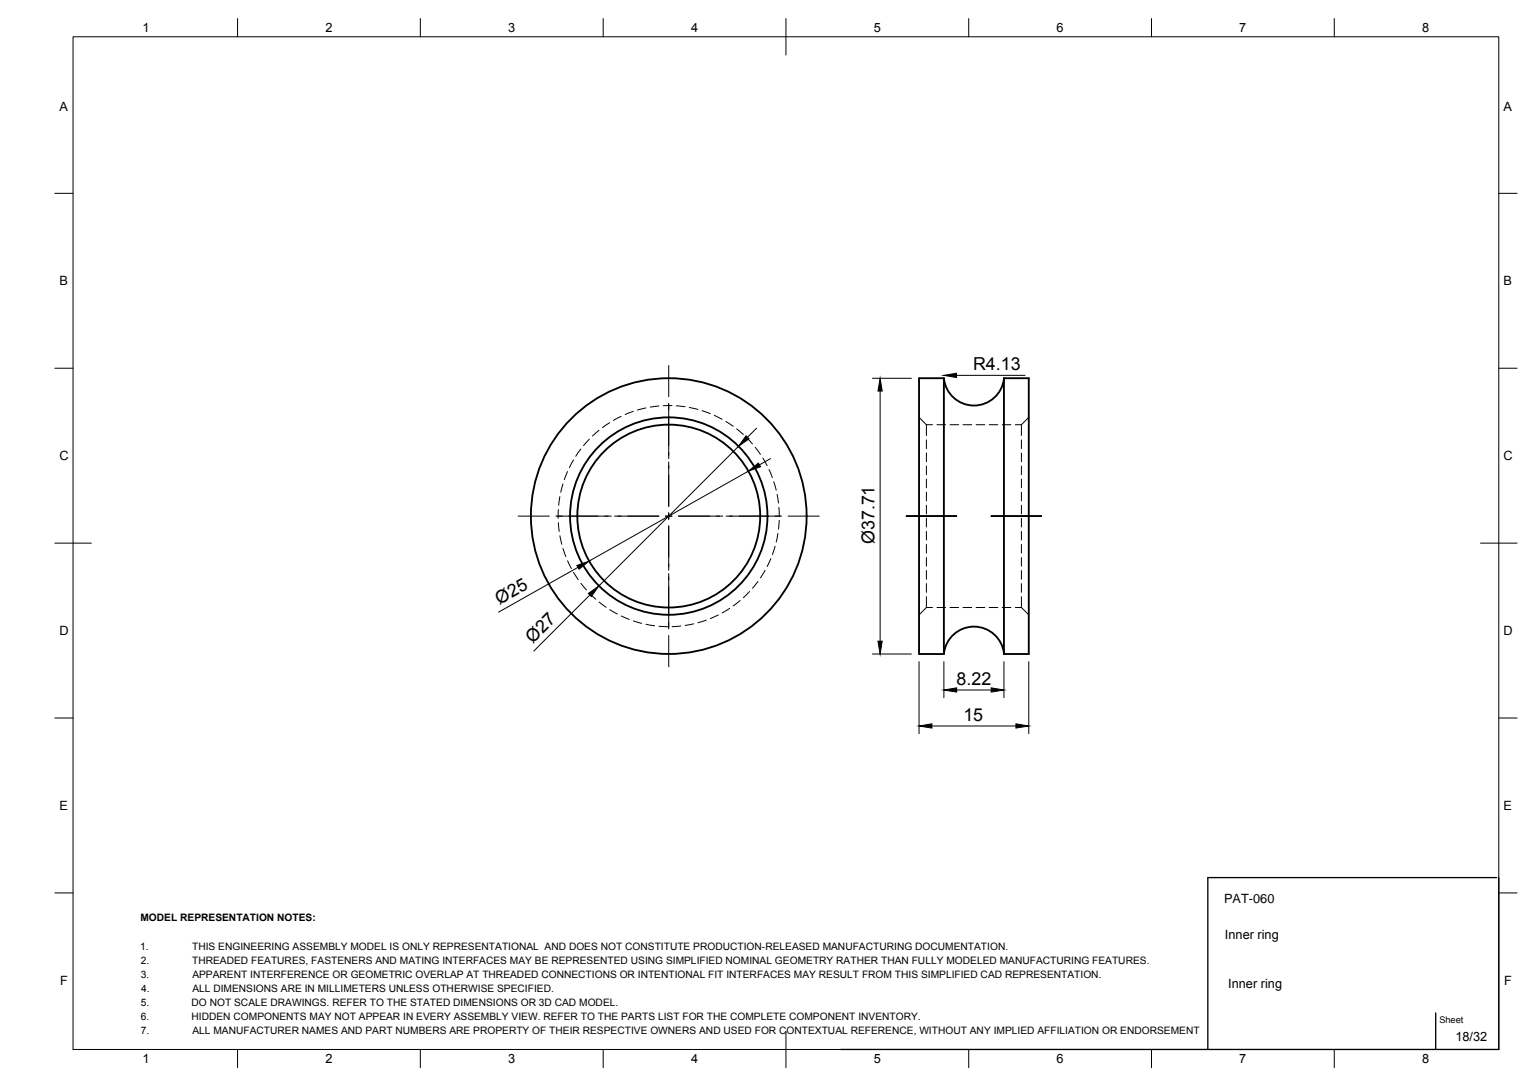
ISO-10303-21;
HEADER;
/* Generated by software containing ST-Developer
 * from STEP Tools, Inc. (www.steptools.com) 
 */

FILE_DESCRIPTION(
/* description */ ('Indexing fixture plate with plunger'),
/* implementation_level */ '2;1');

FILE_NAME(
/* name */ 'Inner ring.step',
/* time_stamp */ '2026-10-28T03:23:41-07:00',
/* author */ (''),
/* organization */ (''),
/* preprocessor_version */ 'ST-DEVELOPER v20.2',
/* originating_system */ 'Autodesk Translation Framework v15.17.0.0',
/* authorisation */ '');

FILE_SCHEMA (('AUTOMOTIVE_DESIGN { 1 0 10303 214 3 1 1 }'));
ENDSEC;

DATA;
#10=MECHANICAL_DESIGN_GEOMETRIC_PRESENTATION_REPRESENTATION('',(#330),#10020);
#213=TOROIDAL_SURFACE('',#5086,1.925,0.412776);
#218=CONICAL_SURFACE('',#5097,1.3,0.785398163397449);
#219=CONICAL_SURFACE('',#5104,1.3,0.785398163397449);
#276=SHAPE_REPRESENTATION_RELATIONSHIP('SRR','None',#10151,#303);
#303=ADVANCED_BREP_SHAPE_REPRESENTATION('',(#365),#10004);
#330=STYLED_ITEM('',(#10368),#365);
#365=MANIFOLD_SOLID_BREP('Body1',#4585);
#431=FACE_BOUND('',#1091,.T.);
#432=FACE_BOUND('',#1094,.T.);
#583=PLANE('',#5099);
#584=PLANE('',#5102);
#756=FACE_OUTER_BOUND('',#1086,.T.);
#757=FACE_OUTER_BOUND('',#1087,.T.);
#758=FACE_OUTER_BOUND('',#1088,.T.);
#759=FACE_OUTER_BOUND('',#1089,.T.);
#760=FACE_OUTER_BOUND('',#1090,.T.);
#761=FACE_OUTER_BOUND('',#1092,.T.);
#762=FACE_OUTER_BOUND('',#1093,.T.);
#763=FACE_OUTER_BOUND('',#1095,.T.);
#1086=EDGE_LOOP('',(#3371,#3372,#3373,#3374,#3375,#3376));
#1087=EDGE_LOOP('',(#3377,#3378,#3379,#3380,#3381));
#1088=EDGE_LOOP('',(#3382,#3383,#3384,#3385));
#1089=EDGE_LOOP('',(#3386,#3387,#3388,#3389));
#1090=EDGE_LOOP('',(#3390));
#1091=EDGE_LOOP('',(#3391));
#1092=EDGE_LOOP('',(#3392,#3393,#3394,#3395,#3396));
#1093=EDGE_LOOP('',(#3397));
#1094=EDGE_LOOP('',(#3398));
#1095=EDGE_LOOP('',(#3399,#3400,#3401,#3402));
#1463=LINE('',#8611,#1683);
#1464=LINE('',#8617,#1684);
#1465=LINE('',#8621,#1685);
#1466=LINE('',#8627,#1686);
#1467=LINE('',#8632,#1687);
#1683=VECTOR('',#6016,1.88531);
#1684=VECTOR('',#6023,1.25);
#1685=VECTOR('',#6028,1.3);
#1686=VECTOR('',#6037,1.88531);
#1687=VECTOR('',#6044,1.3);
#1909=CIRCLE('',#5087,1.88531);
#1910=CIRCLE('',#5088,1.88531);
#1911=CIRCLE('',#5089,0.412776);
#1912=CIRCLE('',#5090,1.88531);
#1913=CIRCLE('',#5091,1.88531);
#1914=CIRCLE('',#5093,1.88531);
#1915=CIRCLE('',#5095,1.25);
#1916=CIRCLE('',#5096,1.25);
#1917=CIRCLE('',#5098,1.35);
#1918=CIRCLE('',#5101,1.88531);
#1919=CIRCLE('',#5103,1.35);
#2237=VERTEX_POINT('',#8600);
#2238=VERTEX_POINT('',#8601);
#2239=VERTEX_POINT('',#8604);
#2240=VERTEX_POINT('',#8606);
#2241=VERTEX_POINT('',#8610);
#2242=VERTEX_POINT('',#8614);
#2243=VERTEX_POINT('',#8616);
#2244=VERTEX_POINT('',#8620);
#2245=VERTEX_POINT('',#8625);
#2246=VERTEX_POINT('',#8629);
#2665=EDGE_CURVE('',#2237,#2238,#1909,.T.);
#2666=EDGE_CURVE('',#2238,#2237,#1910,.T.);
#2667=EDGE_CURVE('',#2238,#2239,#1911,.T.);
#2668=EDGE_CURVE('',#2240,#2239,#1912,.T.);
#2669=EDGE_CURVE('',#2239,#2240,#1913,.T.);
#2670=EDGE_CURVE('',#2240,#2241,#1463,.T.);
#2671=EDGE_CURVE('',#2241,#2241,#1914,.T.);
#2672=EDGE_CURVE('',#2242,#2242,#1915,.T.);
#2673=EDGE_CURVE('',#2242,#2243,#1464,.T.);
#2674=EDGE_CURVE('',#2243,#2243,#1916,.T.);
#2675=EDGE_CURVE('',#2243,#2244,#1465,.T.);
#2676=EDGE_CURVE('',#2244,#2244,#1917,.T.);
#2677=EDGE_CURVE('',#2245,#2245,#1918,.T.);
#2678=EDGE_CURVE('',#2245,#2237,#1466,.T.);
#2679=EDGE_CURVE('',#2246,#2246,#1919,.T.);
#2680=EDGE_CURVE('',#2246,#2242,#1467,.T.);
#3371=ORIENTED_EDGE('',*,*,#2665,.F.);
#3372=ORIENTED_EDGE('',*,*,#2666,.F.);
#3373=ORIENTED_EDGE('',*,*,#2667,.T.);
#3374=ORIENTED_EDGE('',*,*,#2668,.F.);
#3375=ORIENTED_EDGE('',*,*,#2669,.F.);
#3376=ORIENTED_EDGE('',*,*,#2667,.F.);
#3377=ORIENTED_EDGE('',*,*,#2668,.T.);
#3378=ORIENTED_EDGE('',*,*,#2669,.T.);
#3379=ORIENTED_EDGE('',*,*,#2670,.T.);
#3380=ORIENTED_EDGE('',*,*,#2671,.T.);
#3381=ORIENTED_EDGE('',*,*,#2670,.F.);
#3382=ORIENTED_EDGE('',*,*,#2672,.T.);
#3383=ORIENTED_EDGE('',*,*,#2673,.T.);
#3384=ORIENTED_EDGE('',*,*,#2674,.F.);
#3385=ORIENTED_EDGE('',*,*,#2673,.F.);
#3386=ORIENTED_EDGE('',*,*,#2674,.T.);
#3387=ORIENTED_EDGE('',*,*,#2675,.T.);
#3388=ORIENTED_EDGE('',*,*,#2676,.F.);
#3389=ORIENTED_EDGE('',*,*,#2675,.F.);
#3390=ORIENTED_EDGE('',*,*,#2671,.F.);
#3391=ORIENTED_EDGE('',*,*,#2676,.T.);
#3392=ORIENTED_EDGE('',*,*,#2677,.F.);
#3393=ORIENTED_EDGE('',*,*,#2678,.T.);
#3394=ORIENTED_EDGE('',*,*,#2665,.T.);
#3395=ORIENTED_EDGE('',*,*,#2666,.T.);
#3396=ORIENTED_EDGE('',*,*,#2678,.F.);
#3397=ORIENTED_EDGE('',*,*,#2677,.T.);
#3398=ORIENTED_EDGE('',*,*,#2679,.F.);
#3399=ORIENTED_EDGE('',*,*,#2679,.T.);
#3400=ORIENTED_EDGE('',*,*,#2680,.T.);
#3401=ORIENTED_EDGE('',*,*,#2672,.F.);
#3402=ORIENTED_EDGE('',*,*,#2680,.F.);
#4203=CYLINDRICAL_SURFACE('',#5092,1.88531);
#4204=CYLINDRICAL_SURFACE('',#5094,1.25);
#4205=CYLINDRICAL_SURFACE('',#5100,1.88531);
#4371=ADVANCED_FACE('',(#756),#213,.F.);
#4372=ADVANCED_FACE('',(#757),#4203,.T.);
#4373=ADVANCED_FACE('',(#758),#4204,.F.);
#4374=ADVANCED_FACE('',(#759),#218,.F.);
#4375=ADVANCED_FACE('',(#760,#431),#583,.T.);
#4376=ADVANCED_FACE('',(#761),#4205,.T.);
#4377=ADVANCED_FACE('',(#762,#432),#584,.T.);
#4378=ADVANCED_FACE('',(#763),#219,.F.);
#4585=CLOSED_SHELL('',(#4371,#4372,#4373,#4374,#4375,#4376,#4377,#4378));
#5085=AXIS2_PLACEMENT_3D('',#8598,#6000,#6001);
#5086=AXIS2_PLACEMENT_3D('',#8599,#6002,#6003);
#5087=AXIS2_PLACEMENT_3D('',#8602,#6004,#6005);
#5088=AXIS2_PLACEMENT_3D('',#8603,#6006,#6007);
#5089=AXIS2_PLACEMENT_3D('',#8605,#6008,#6009);
#5090=AXIS2_PLACEMENT_3D('',#8607,#6010,#6011);
#5091=AXIS2_PLACEMENT_3D('',#8608,#6012,#6013);
#5092=AXIS2_PLACEMENT_3D('',#8609,#6014,#6015);
#5093=AXIS2_PLACEMENT_3D('',#8612,#6017,#6018);
#5094=AXIS2_PLACEMENT_3D('',#8613,#6019,#6020);
#5095=AXIS2_PLACEMENT_3D('',#8615,#6021,#6022);
#5096=AXIS2_PLACEMENT_3D('',#8618,#6024,#6025);
#5097=AXIS2_PLACEMENT_3D('',#8619,#6026,#6027);
#5098=AXIS2_PLACEMENT_3D('',#8622,#6029,#6030);
#5099=AXIS2_PLACEMENT_3D('',#8623,#6031,#6032);
#5100=AXIS2_PLACEMENT_3D('',#8624,#6033,#6034);
#5101=AXIS2_PLACEMENT_3D('',#8626,#6035,#6036);
#5102=AXIS2_PLACEMENT_3D('',#8628,#6038,#6039);
#5103=AXIS2_PLACEMENT_3D('',#8630,#6040,#6041);
#5104=AXIS2_PLACEMENT_3D('',#8631,#6042,#6043);
#6000=DIRECTION('axis',(0.,0.,1.));
#6001=DIRECTION('refdir',(1.,0.,0.));
#6002=DIRECTION('center_axis',(0.,-1.,0.));
#6003=DIRECTION('ref_axis',(0.,0.,-1.));
#6004=DIRECTION('center_axis',(0.,-1.,0.));
#6005=DIRECTION('ref_axis',(1.,0.,0.));
#6006=DIRECTION('center_axis',(0.,-1.,0.));
#6007=DIRECTION('ref_axis',(1.,0.,0.));
#6008=DIRECTION('center_axis',(1.,0.,1.22464679914735E-16));
#6009=DIRECTION('ref_axis',(-1.22464679914735E-16,0.,1.));
#6010=DIRECTION('center_axis',(0.,1.,0.));
#6011=DIRECTION('ref_axis',(1.,0.,0.));
#6012=DIRECTION('center_axis',(0.,1.,0.));
#6013=DIRECTION('ref_axis',(1.,0.,0.));
#6014=DIRECTION('center_axis',(0.,-1.,0.));
#6015=DIRECTION('ref_axis',(1.,0.,0.));
#6016=DIRECTION('',(0.,1.,0.));
#6017=DIRECTION('center_axis',(0.,-1.,0.));
#6018=DIRECTION('ref_axis',(1.,0.,0.));
#6019=DIRECTION('center_axis',(0.,-1.,0.));
#6020=DIRECTION('ref_axis',(1.,0.,0.));
#6021=DIRECTION('center_axis',(0.,-1.,0.));
#6022=DIRECTION('ref_axis',(1.,0.,0.));
#6023=DIRECTION('',(0.,1.,0.));
#6024=DIRECTION('center_axis',(0.,-1.,0.));
#6025=DIRECTION('ref_axis',(1.,0.,0.));
#6026=DIRECTION('center_axis',(0.,1.,0.));
#6027=DIRECTION('ref_axis',(1.,0.,0.));
#6028=DIRECTION('',(-0.707106781186548,0.707106781186547,-8.65956056235494E-17));
#6029=DIRECTION('center_axis',(0.,-1.,0.));
#6030=DIRECTION('ref_axis',(1.,0.,0.));
#6031=DIRECTION('center_axis',(0.,1.,0.));
#6032=DIRECTION('ref_axis',(0.,0.,1.));
#6033=DIRECTION('center_axis',(0.,-1.,0.));
#6034=DIRECTION('ref_axis',(1.,0.,0.));
#6035=DIRECTION('center_axis',(0.,-1.,0.));
#6036=DIRECTION('ref_axis',(1.,0.,0.));
#6037=DIRECTION('',(0.,1.,0.));
#6038=DIRECTION('center_axis',(0.,-1.,0.));
#6039=DIRECTION('ref_axis',(0.,0.,-1.));
#6040=DIRECTION('center_axis',(0.,-1.,0.));
#6041=DIRECTION('ref_axis',(1.,0.,0.));
#6042=DIRECTION('center_axis',(0.,-1.,0.));
#6043=DIRECTION('ref_axis',(1.,0.,0.));
#6044=DIRECTION('',(0.707106781186548,0.707106781186547,8.65956056235494E-17));
#8598=CARTESIAN_POINT('',(0.,0.,0.));
#8599=CARTESIAN_POINT('Origin',(0.,0.,0.));
#8600=CARTESIAN_POINT('',(-1.88531,-0.410863395882378,-2.3088388569005E-16));
#8601=CARTESIAN_POINT('',(-2.3088388569005E-16,-0.410863395882378,1.88531));
#8602=CARTESIAN_POINT('Origin',(0.,-0.410863395882378,0.));
#8603=CARTESIAN_POINT('Origin',(0.,-0.410863395882378,0.));
#8604=CARTESIAN_POINT('',(-2.3088388569005E-16,0.410863395882378,1.88531));
#8605=CARTESIAN_POINT('Origin',(-2.35744508835865E-16,0.,1.925));
#8606=CARTESIAN_POINT('',(-1.88531,0.410863395882378,2.3088388569005E-16));
#8607=CARTESIAN_POINT('Origin',(0.,0.410863395882378,0.));
#8608=CARTESIAN_POINT('Origin',(0.,0.410863395882378,0.));
#8609=CARTESIAN_POINT('Origin',(0.,0.,0.));
#8610=CARTESIAN_POINT('',(-1.88531,0.75,-2.3088388569005E-16));
#8611=CARTESIAN_POINT('',(-1.88531,0.,-2.3088388569005E-16));
#8612=CARTESIAN_POINT('Origin',(0.,0.75,0.));
#8613=CARTESIAN_POINT('Origin',(0.,0.,0.));
#8614=CARTESIAN_POINT('',(-1.25,-0.65,-1.53080849893419E-16));
#8615=CARTESIAN_POINT('Origin',(0.,-0.65,0.));
#8616=CARTESIAN_POINT('',(-1.25,0.65,-1.53080849893419E-16));
#8617=CARTESIAN_POINT('',(-1.25,0.,-1.53080849893419E-16));
#8618=CARTESIAN_POINT('Origin',(0.,0.65,0.));
#8619=CARTESIAN_POINT('Origin',(0.,0.7,0.));
#8620=CARTESIAN_POINT('',(-1.35,0.75,-1.65327317884893E-16));
#8621=CARTESIAN_POINT('',(-1.3,0.7,-1.59204083889156E-16));
#8622=CARTESIAN_POINT('Origin',(0.,0.75,0.));
#8623=CARTESIAN_POINT('Origin',(1.88531,0.75,0.));
#8624=CARTESIAN_POINT('Origin',(0.,0.,0.));
#8625=CARTESIAN_POINT('',(-1.88531,-0.75,-2.3088388569005E-16));
#8626=CARTESIAN_POINT('Origin',(0.,-0.75,0.));
#8627=CARTESIAN_POINT('',(-1.88531,0.,-2.3088388569005E-16));
#8628=CARTESIAN_POINT('Origin',(1.35,-0.75,0.));
#8629=CARTESIAN_POINT('',(-1.35,-0.75,-1.65327317884893E-16));
#8630=CARTESIAN_POINT('Origin',(0.,-0.75,0.));
#8631=CARTESIAN_POINT('Origin',(0.,-0.7,0.));
#8632=CARTESIAN_POINT('',(-1.3,-0.7,-1.59204083889156E-16));
#9971=UNCERTAINTY_MEASURE_WITH_UNIT(LENGTH_MEASURE(0.001),#10021,
'DISTANCE_ACCURACY_VALUE',
'Maximum model space distance between geometric entities at asserted c
onnectivities');
#9987=UNCERTAINTY_MEASURE_WITH_UNIT(LENGTH_MEASURE(0.001),#10021,
'DISTANCE_ACCURACY_VALUE',
'Maximum model space distance between geometric entities at asserted c
onnectivities');
#10004=(
GEOMETRIC_REPRESENTATION_CONTEXT(3)
GLOBAL_UNCERTAINTY_ASSIGNED_CONTEXT((#9971))
GLOBAL_UNIT_ASSIGNED_CONTEXT((#10021,#10023,#10024))
REPRESENTATION_CONTEXT('','3D')
);
#10020=(
GEOMETRIC_REPRESENTATION_CONTEXT(3)
GLOBAL_UNCERTAINTY_ASSIGNED_CONTEXT((#9987))
GLOBAL_UNIT_ASSIGNED_CONTEXT((#10021,#10023,#10024))
REPRESENTATION_CONTEXT('','3D')
);
#10021=(
LENGTH_UNIT()
NAMED_UNIT(*)
SI_UNIT(.CENTI.,.METRE.)
);
#10023=(
NAMED_UNIT(*)
PLANE_ANGLE_UNIT()
SI_UNIT($,.RADIAN.)
);
#10024=(
NAMED_UNIT(*)
SI_UNIT($,.STERADIAN.)
SOLID_ANGLE_UNIT()
);
#10041=SHAPE_DEFINITION_REPRESENTATION(#10073,#10151);
#10073=PRODUCT_DEFINITION_SHAPE('',$,#10184);
#10151=SHAPE_REPRESENTATION('',(#5085),#10004);
#10167=PRODUCT_DEFINITION_CONTEXT('part definition',#10265,'design');
#10184=PRODUCT_DEFINITION('Inner ring','Inner ring',#10216,#10167);
#10216=PRODUCT_DEFINITION_FORMATION('',$,#10283);
#10265=APPLICATION_CONTEXT(
'Core Data for Automotive Mechanical Design Process');
#10266=PRODUCT_CONTEXT('part definition',#10265,'mechanical');
#10283=PRODUCT('Inner ring','Inner ring','Inner ring',(#10266));
#10362=COLOUR_RGB('Grey',0.48,0.52,0.57);
#10363=FILL_AREA_STYLE_COLOUR('',#10362);
#10364=FILL_AREA_STYLE('',(#10363));
#10365=SURFACE_STYLE_FILL_AREA(#10364);
#10366=SURFACE_SIDE_STYLE('',(#10365));
#10367=SURFACE_STYLE_USAGE(.BOTH.,#10366);
#10368=PRESENTATION_STYLE_ASSIGNMENT((#10367));
ENDSEC;
END-ISO-10303-21;
